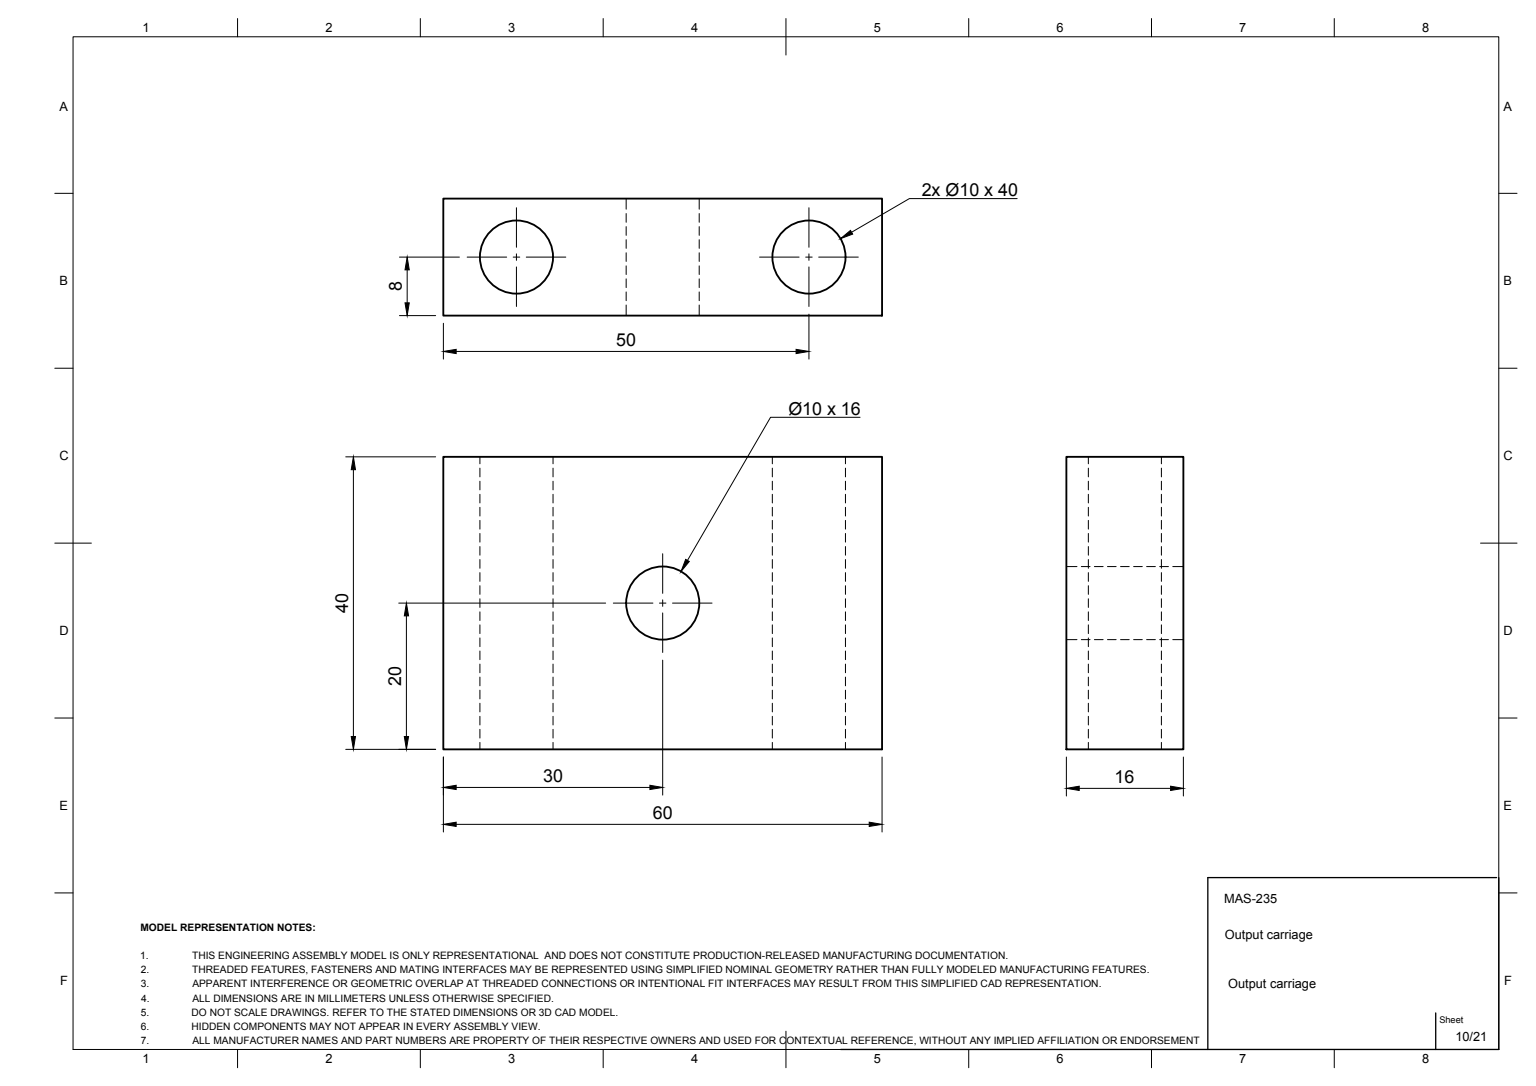
ISO-10303-21;
HEADER;
/* Generated by software containing ST-Developer
 * from STEP Tools, Inc. (www.steptools.com) 
 */

FILE_DESCRIPTION(
/* description */ ('Independent Whitworth quick-return mechanism. Crank radius40, ground-
center spacing80, lever180, connecting rod160, output guide X200. Nomi
nal stroke180 and long/short phase ratio2. Retained guide rods, replac
eable bearing sleeves and captured sliding shoe. No load or production
 rating assigned.'),
/* implementation_level */ '2;1');

FILE_NAME(
/* name */ 'Output carriage.step',
/* time_stamp */ '2026-11-09T18:22:56-08:00',
/* author */ (''),
/* organization */ (''),
/* preprocessor_version */ 'ST-DEVELOPER v20.2',
/* originating_system */ 'Autodesk Translation Framework v15.17.0.0',
/* authorisation */ '');

FILE_SCHEMA (('AUTOMOTIVE_DESIGN { 1 0 10303 214 3 1 1 }'));
ENDSEC;

DATA;
#10=MECHANICAL_DESIGN_GEOMETRIC_PRESENTATION_REPRESENTATION('',(#226),#4388);
#186=SHAPE_REPRESENTATION_RELATIONSHIP('SRR','None',#4485,#206);
#206=ADVANCED_BREP_SHAPE_REPRESENTATION('',(#246),#4375);
#226=STYLED_ITEM('',(#4593),#246);
#246=MANIFOLD_SOLID_BREP('Body1',#2331);
#283=FACE_BOUND('',#631,.T.);
#284=FACE_BOUND('',#632,.T.);
#285=FACE_BOUND('',#635,.T.);
#286=FACE_BOUND('',#636,.T.);
#287=FACE_BOUND('',#639,.T.);
#288=FACE_BOUND('',#641,.T.);
#349=PLANE('',#2676);
#350=PLANE('',#2677);
#351=PLANE('',#2678);
#352=PLANE('',#2679);
#353=PLANE('',#2680);
#354=PLANE('',#2681);
#456=FACE_OUTER_BOUND('',#627,.T.);
#457=FACE_OUTER_BOUND('',#628,.T.);
#458=FACE_OUTER_BOUND('',#629,.T.);
#459=FACE_OUTER_BOUND('',#630,.T.);
#460=FACE_OUTER_BOUND('',#633,.T.);
#461=FACE_OUTER_BOUND('',#634,.T.);
#462=FACE_OUTER_BOUND('',#637,.T.);
#463=FACE_OUTER_BOUND('',#638,.T.);
#464=FACE_OUTER_BOUND('',#640,.T.);
#627=EDGE_LOOP('',(#1816,#1817,#1818,#1819));
#628=EDGE_LOOP('',(#1820,#1821,#1822,#1823));
#629=EDGE_LOOP('',(#1824,#1825,#1826,#1827));
#630=EDGE_LOOP('',(#1828,#1829,#1830,#1831));
#631=EDGE_LOOP('',(#1832));
#632=EDGE_LOOP('',(#1833));
#633=EDGE_LOOP('',(#1834,#1835,#1836,#1837));
#634=EDGE_LOOP('',(#1838,#1839,#1840,#1841));
#635=EDGE_LOOP('',(#1842));
#636=EDGE_LOOP('',(#1843));
#637=EDGE_LOOP('',(#1844,#1845,#1846,#1847));
#638=EDGE_LOOP('',(#1848,#1849,#1850,#1851));
#639=EDGE_LOOP('',(#1852));
#640=EDGE_LOOP('',(#1853,#1854,#1855,#1856));
#641=EDGE_LOOP('',(#1857));
#828=LINE('',#3949,#967);
#829=LINE('',#3955,#968);
#830=LINE('',#3961,#969);
#831=LINE('',#3966,#970);
#832=LINE('',#3968,#971);
#833=LINE('',#3970,#972);
#834=LINE('',#3971,#973);
#835=LINE('',#3974,#974);
#836=LINE('',#3976,#975);
#837=LINE('',#3977,#976);
#838=LINE('',#3980,#977);
#839=LINE('',#3982,#978);
#840=LINE('',#3983,#979);
#841=LINE('',#3985,#980);
#842=LINE('',#3986,#981);
#967=VECTOR('',#3174,5.);
#968=VECTOR('',#3181,5.);
#969=VECTOR('',#3188,5.);
#970=VECTOR('',#3193,10.);
#971=VECTOR('',#3194,10.);
#972=VECTOR('',#3195,10.);
#973=VECTOR('',#3196,10.);
#974=VECTOR('',#3199,10.);
#975=VECTOR('',#3200,10.);
#976=VECTOR('',#3201,10.);
#977=VECTOR('',#3204,10.);
#978=VECTOR('',#3205,10.);
#979=VECTOR('',#3206,10.);
#980=VECTOR('',#3209,10.);
#981=VECTOR('',#3210,10.);
#1079=CIRCLE('',#2668,5.);
#1080=CIRCLE('',#2669,5.);
#1081=CIRCLE('',#2671,5.);
#1082=CIRCLE('',#2672,5.);
#1083=CIRCLE('',#2674,5.);
#1084=CIRCLE('',#2675,5.);
#1233=VERTEX_POINT('',#3946);
#1234=VERTEX_POINT('',#3948);
#1235=VERTEX_POINT('',#3952);
#1236=VERTEX_POINT('',#3954);
#1237=VERTEX_POINT('',#3958);
#1238=VERTEX_POINT('',#3960);
#1239=VERTEX_POINT('',#3964);
#1240=VERTEX_POINT('',#3965);
#1241=VERTEX_POINT('',#3967);
#1242=VERTEX_POINT('',#3969);
#1243=VERTEX_POINT('',#3973);
#1244=VERTEX_POINT('',#3975);
#1245=VERTEX_POINT('',#3979);
#1246=VERTEX_POINT('',#3981);
#1444=EDGE_CURVE('',#1233,#1233,#1079,.T.);
#1445=EDGE_CURVE('',#1233,#1234,#828,.T.);
#1446=EDGE_CURVE('',#1234,#1234,#1080,.T.);
#1447=EDGE_CURVE('',#1235,#1235,#1081,.T.);
#1448=EDGE_CURVE('',#1235,#1236,#829,.T.);
#1449=EDGE_CURVE('',#1236,#1236,#1082,.T.);
#1450=EDGE_CURVE('',#1237,#1237,#1083,.T.);
#1451=EDGE_CURVE('',#1237,#1238,#830,.T.);
#1452=EDGE_CURVE('',#1238,#1238,#1084,.T.);
#1453=EDGE_CURVE('',#1239,#1240,#831,.T.);
#1454=EDGE_CURVE('',#1240,#1241,#832,.T.);
#1455=EDGE_CURVE('',#1242,#1241,#833,.T.);
#1456=EDGE_CURVE('',#1239,#1242,#834,.T.);
#1457=EDGE_CURVE('',#1243,#1239,#835,.T.);
#1458=EDGE_CURVE('',#1244,#1242,#836,.T.);
#1459=EDGE_CURVE('',#1243,#1244,#837,.T.);
#1460=EDGE_CURVE('',#1245,#1243,#838,.T.);
#1461=EDGE_CURVE('',#1246,#1244,#839,.T.);
#1462=EDGE_CURVE('',#1245,#1246,#840,.T.);
#1463=EDGE_CURVE('',#1240,#1245,#841,.T.);
#1464=EDGE_CURVE('',#1241,#1246,#842,.T.);
#1816=ORIENTED_EDGE('',*,*,#1444,.F.);
#1817=ORIENTED_EDGE('',*,*,#1445,.T.);
#1818=ORIENTED_EDGE('',*,*,#1446,.F.);
#1819=ORIENTED_EDGE('',*,*,#1445,.F.);
#1820=ORIENTED_EDGE('',*,*,#1447,.F.);
#1821=ORIENTED_EDGE('',*,*,#1448,.T.);
#1822=ORIENTED_EDGE('',*,*,#1449,.F.);
#1823=ORIENTED_EDGE('',*,*,#1448,.F.);
#1824=ORIENTED_EDGE('',*,*,#1450,.F.);
#1825=ORIENTED_EDGE('',*,*,#1451,.T.);
#1826=ORIENTED_EDGE('',*,*,#1452,.F.);
#1827=ORIENTED_EDGE('',*,*,#1451,.F.);
#1828=ORIENTED_EDGE('',*,*,#1453,.T.);
#1829=ORIENTED_EDGE('',*,*,#1454,.T.);
#1830=ORIENTED_EDGE('',*,*,#1455,.F.);
#1831=ORIENTED_EDGE('',*,*,#1456,.F.);
#1832=ORIENTED_EDGE('',*,*,#1447,.T.);
#1833=ORIENTED_EDGE('',*,*,#1450,.T.);
#1834=ORIENTED_EDGE('',*,*,#1457,.T.);
#1835=ORIENTED_EDGE('',*,*,#1456,.T.);
#1836=ORIENTED_EDGE('',*,*,#1458,.F.);
#1837=ORIENTED_EDGE('',*,*,#1459,.F.);
#1838=ORIENTED_EDGE('',*,*,#1460,.T.);
#1839=ORIENTED_EDGE('',*,*,#1459,.T.);
#1840=ORIENTED_EDGE('',*,*,#1461,.F.);
#1841=ORIENTED_EDGE('',*,*,#1462,.F.);
#1842=ORIENTED_EDGE('',*,*,#1449,.T.);
#1843=ORIENTED_EDGE('',*,*,#1452,.T.);
#1844=ORIENTED_EDGE('',*,*,#1463,.T.);
#1845=ORIENTED_EDGE('',*,*,#1462,.T.);
#1846=ORIENTED_EDGE('',*,*,#1464,.F.);
#1847=ORIENTED_EDGE('',*,*,#1454,.F.);
#1848=ORIENTED_EDGE('',*,*,#1464,.T.);
#1849=ORIENTED_EDGE('',*,*,#1461,.T.);
#1850=ORIENTED_EDGE('',*,*,#1458,.T.);
#1851=ORIENTED_EDGE('',*,*,#1455,.T.);
#1852=ORIENTED_EDGE('',*,*,#1444,.T.);
#1853=ORIENTED_EDGE('',*,*,#1463,.F.);
#1854=ORIENTED_EDGE('',*,*,#1453,.F.);
#1855=ORIENTED_EDGE('',*,*,#1457,.F.);
#1856=ORIENTED_EDGE('',*,*,#1460,.F.);
#1857=ORIENTED_EDGE('',*,*,#1446,.T.);
#2137=CYLINDRICAL_SURFACE('',#2667,5.);
#2138=CYLINDRICAL_SURFACE('',#2670,5.);
#2139=CYLINDRICAL_SURFACE('',#2673,5.);
#2228=ADVANCED_FACE('',(#456),#2137,.F.);
#2229=ADVANCED_FACE('',(#457),#2138,.F.);
#2230=ADVANCED_FACE('',(#458),#2139,.F.);
#2231=ADVANCED_FACE('',(#459,#283,#284),#349,.T.);
#2232=ADVANCED_FACE('',(#460),#350,.T.);
#2233=ADVANCED_FACE('',(#461,#285,#286),#351,.T.);
#2234=ADVANCED_FACE('',(#462),#352,.T.);
#2235=ADVANCED_FACE('',(#463,#287),#353,.T.);
#2236=ADVANCED_FACE('',(#464,#288),#354,.F.);
#2331=CLOSED_SHELL('',(#2228,#2229,#2230,#2231,#2232,#2233,#2234,#2235,
#2236));
#2666=AXIS2_PLACEMENT_3D('',#3944,#3168,#3169);
#2667=AXIS2_PLACEMENT_3D('',#3945,#3170,#3171);
#2668=AXIS2_PLACEMENT_3D('',#3947,#3172,#3173);
#2669=AXIS2_PLACEMENT_3D('',#3950,#3175,#3176);
#2670=AXIS2_PLACEMENT_3D('',#3951,#3177,#3178);
#2671=AXIS2_PLACEMENT_3D('',#3953,#3179,#3180);
#2672=AXIS2_PLACEMENT_3D('',#3956,#3182,#3183);
#2673=AXIS2_PLACEMENT_3D('',#3957,#3184,#3185);
#2674=AXIS2_PLACEMENT_3D('',#3959,#3186,#3187);
#2675=AXIS2_PLACEMENT_3D('',#3962,#3189,#3190);
#2676=AXIS2_PLACEMENT_3D('',#3963,#3191,#3192);
#2677=AXIS2_PLACEMENT_3D('',#3972,#3197,#3198);
#2678=AXIS2_PLACEMENT_3D('',#3978,#3202,#3203);
#2679=AXIS2_PLACEMENT_3D('',#3984,#3207,#3208);
#2680=AXIS2_PLACEMENT_3D('',#3987,#3211,#3212);
#2681=AXIS2_PLACEMENT_3D('',#3988,#3213,#3214);
#3168=DIRECTION('axis',(0.,0.,1.));
#3169=DIRECTION('refdir',(1.,0.,0.));
#3170=DIRECTION('center_axis',(0.,0.,-1.));
#3171=DIRECTION('ref_axis',(1.,0.,0.));
#3172=DIRECTION('center_axis',(0.,0.,-1.));
#3173=DIRECTION('ref_axis',(1.,0.,0.));
#3174=DIRECTION('',(0.,0.,-1.));
#3175=DIRECTION('center_axis',(0.,0.,1.));
#3176=DIRECTION('ref_axis',(1.,0.,0.));
#3177=DIRECTION('center_axis',(0.,-1.,0.));
#3178=DIRECTION('ref_axis',(0.,0.,1.));
#3179=DIRECTION('center_axis',(0.,-1.,0.));
#3180=DIRECTION('ref_axis',(0.,0.,1.));
#3181=DIRECTION('',(0.,-1.,0.));
#3182=DIRECTION('center_axis',(0.,1.,0.));
#3183=DIRECTION('ref_axis',(0.,0.,1.));
#3184=DIRECTION('center_axis',(0.,-1.,0.));
#3185=DIRECTION('ref_axis',(0.,0.,1.));
#3186=DIRECTION('center_axis',(0.,-1.,0.));
#3187=DIRECTION('ref_axis',(0.,0.,1.));
#3188=DIRECTION('',(0.,-1.,0.));
#3189=DIRECTION('center_axis',(0.,1.,0.));
#3190=DIRECTION('ref_axis',(0.,0.,1.));
#3191=DIRECTION('center_axis',(0.,1.,0.));
#3192=DIRECTION('ref_axis',(-1.,0.,0.));
#3193=DIRECTION('',(-1.,0.,0.));
#3194=DIRECTION('',(0.,0.,1.));
#3195=DIRECTION('',(-1.,0.,0.));
#3196=DIRECTION('',(0.,0.,1.));
#3197=DIRECTION('center_axis',(1.,0.,0.));
#3198=DIRECTION('ref_axis',(0.,1.,0.));
#3199=DIRECTION('',(0.,1.,0.));
#3200=DIRECTION('',(0.,1.,0.));
#3201=DIRECTION('',(0.,0.,1.));
#3202=DIRECTION('center_axis',(0.,-1.,0.));
#3203=DIRECTION('ref_axis',(1.,0.,0.));
#3204=DIRECTION('',(1.,0.,0.));
#3205=DIRECTION('',(1.,0.,0.));
#3206=DIRECTION('',(0.,0.,1.));
#3207=DIRECTION('center_axis',(-1.,0.,0.));
#3208=DIRECTION('ref_axis',(0.,-1.,0.));
#3209=DIRECTION('',(0.,-1.,0.));
#3210=DIRECTION('',(0.,-1.,0.));
#3211=DIRECTION('center_axis',(0.,0.,1.));
#3212=DIRECTION('ref_axis',(1.,0.,0.));
#3213=DIRECTION('center_axis',(0.,0.,1.));
#3214=DIRECTION('ref_axis',(1.,0.,0.));
#3944=CARTESIAN_POINT('',(0.,0.,0.));
#3945=CARTESIAN_POINT('Origin',(0.,0.,8.));
#3946=CARTESIAN_POINT('',(-5.,6.12323399573677E-16,16.));
#3947=CARTESIAN_POINT('Origin',(0.,0.,16.));
#3948=CARTESIAN_POINT('',(-5.,6.12323399573677E-16,0.));
#3949=CARTESIAN_POINT('',(-5.,6.12323399573677E-16,8.));
#3950=CARTESIAN_POINT('Origin',(0.,0.,0.));
#3951=CARTESIAN_POINT('Origin',(-20.,0.,8.));
#3952=CARTESIAN_POINT('',(-20.,20.,3.));
#3953=CARTESIAN_POINT('Origin',(-20.,20.,8.));
#3954=CARTESIAN_POINT('',(-20.,-20.,3.));
#3955=CARTESIAN_POINT('',(-20.,0.,3.));
#3956=CARTESIAN_POINT('Origin',(-20.,-20.,8.));
#3957=CARTESIAN_POINT('Origin',(20.,0.,8.));
#3958=CARTESIAN_POINT('',(20.,20.,3.));
#3959=CARTESIAN_POINT('Origin',(20.,20.,8.));
#3960=CARTESIAN_POINT('',(20.,-20.,3.));
#3961=CARTESIAN_POINT('',(20.,0.,3.));
#3962=CARTESIAN_POINT('Origin',(20.,-20.,8.));
#3963=CARTESIAN_POINT('Origin',(30.,20.,0.));
#3964=CARTESIAN_POINT('',(30.,20.,0.));
#3965=CARTESIAN_POINT('',(-30.,20.,0.));
#3966=CARTESIAN_POINT('',(30.,20.,0.));
#3967=CARTESIAN_POINT('',(-30.,20.,16.));
#3968=CARTESIAN_POINT('',(-30.,20.,0.));
#3969=CARTESIAN_POINT('',(30.,20.,16.));
#3970=CARTESIAN_POINT('',(30.,20.,16.));
#3971=CARTESIAN_POINT('',(30.,20.,0.));
#3972=CARTESIAN_POINT('Origin',(30.,-20.,0.));
#3973=CARTESIAN_POINT('',(30.,-20.,0.));
#3974=CARTESIAN_POINT('',(30.,-20.,0.));
#3975=CARTESIAN_POINT('',(30.,-20.,16.));
#3976=CARTESIAN_POINT('',(30.,-20.,16.));
#3977=CARTESIAN_POINT('',(30.,-20.,0.));
#3978=CARTESIAN_POINT('Origin',(-30.,-20.,0.));
#3979=CARTESIAN_POINT('',(-30.,-20.,0.));
#3980=CARTESIAN_POINT('',(-30.,-20.,0.));
#3981=CARTESIAN_POINT('',(-30.,-20.,16.));
#3982=CARTESIAN_POINT('',(-30.,-20.,16.));
#3983=CARTESIAN_POINT('',(-30.,-20.,0.));
#3984=CARTESIAN_POINT('Origin',(-30.,20.,0.));
#3985=CARTESIAN_POINT('',(-30.,20.,0.));
#3986=CARTESIAN_POINT('',(-30.,20.,16.));
#3987=CARTESIAN_POINT('Origin',(0.,0.,16.));
#3988=CARTESIAN_POINT('Origin',(0.,0.,0.));
#4353=UNCERTAINTY_MEASURE_WITH_UNIT(LENGTH_MEASURE(0.01),#4389,
'DISTANCE_ACCURACY_VALUE',
'Maximum model space distance between geometric entities at asserted c
onnectivities');
#4366=UNCERTAINTY_MEASURE_WITH_UNIT(LENGTH_MEASURE(0.01),#4389,
'DISTANCE_ACCURACY_VALUE',
'Maximum model space distance between geometric entities at asserted c
onnectivities');
#4375=(
GEOMETRIC_REPRESENTATION_CONTEXT(3)
GLOBAL_UNCERTAINTY_ASSIGNED_CONTEXT((#4353))
GLOBAL_UNIT_ASSIGNED_CONTEXT((#4389,#4391,#4392))
REPRESENTATION_CONTEXT('','3D')
);
#4388=(
GEOMETRIC_REPRESENTATION_CONTEXT(3)
GLOBAL_UNCERTAINTY_ASSIGNED_CONTEXT((#4366))
GLOBAL_UNIT_ASSIGNED_CONTEXT((#4389,#4391,#4392))
REPRESENTATION_CONTEXT('','3D')
);
#4389=(
LENGTH_UNIT()
NAMED_UNIT(*)
SI_UNIT(.MILLI.,.METRE.)
);
#4391=(
NAMED_UNIT(*)
PLANE_ANGLE_UNIT()
SI_UNIT($,.RADIAN.)
);
#4392=(
NAMED_UNIT(*)
SI_UNIT($,.STERADIAN.)
SOLID_ANGLE_UNIT()
);
#4401=SHAPE_DEFINITION_REPRESENTATION(#4422,#4485);
#4422=PRODUCT_DEFINITION_SHAPE('',$,#4507);
#4485=SHAPE_REPRESENTATION('',(#2666),#4375);
#4498=PRODUCT_DEFINITION_CONTEXT('part definition',#4563,'design');
#4507=PRODUCT_DEFINITION('Output carriage','Output carriage',#4528,#4498);
#4528=PRODUCT_DEFINITION_FORMATION('',$,#4573);
#4563=APPLICATION_CONTEXT(
'Core Data for Automotive Mechanical Design Process');
#4564=PRODUCT_CONTEXT('part definition',#4563,'mechanical');
#4573=PRODUCT('Output carriage','Output carriage',$,(#4564));
#4593=PRESENTATION_STYLE_ASSIGNMENT((#4607));
#4607=SURFACE_STYLE_USAGE(.BOTH.,#4621);
#4621=SURFACE_SIDE_STYLE('',(#4635));
#4635=SURFACE_STYLE_FILL_AREA(#4649);
#4649=FILL_AREA_STYLE('Dark blue',(#4663));
#4663=FILL_AREA_STYLE_COLOUR('Dark blue',#4677);
#4677=COLOUR_RGB('Dark blue',0.0901960784313725,0.270588235294118,0.513725490196078);
ENDSEC;
END-ISO-10303-21;
